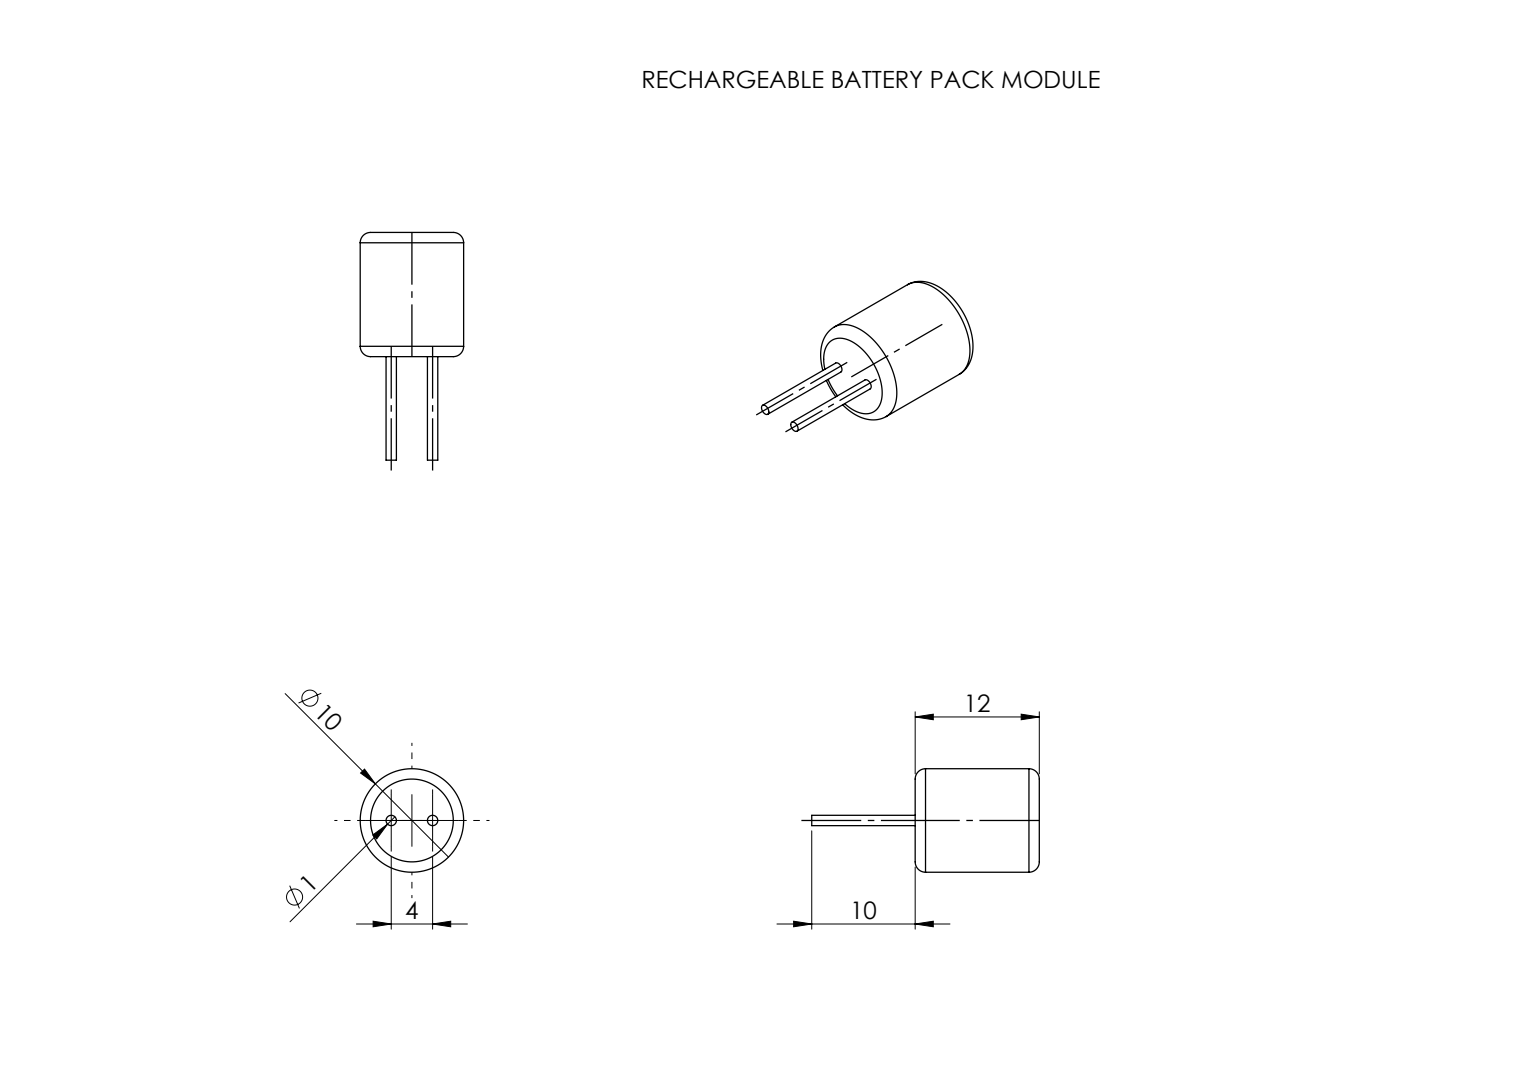
ISO-10303-21;
HEADER;
FILE_DESCRIPTION (('STEP AP214'),
    '1' );
FILE_NAME ('Rechargeable Battery Pack Module.step',
    '2026-10-02T09:26:43',
    ( '' ),
    ( '' ),
    'SwSTEP 2.0',
    'SolidWorks 2026',
    '' );
FILE_SCHEMA (( 'AUTOMOTIVE_DESIGN' ));
ENDSEC;

DATA;
#746=ORIENTED_EDGE ( 'NONE', *, *, #80621, .T. ) ;
#776=VERTEX_POINT ( 'NONE', #34676 ) ;
#917=CYLINDRICAL_SURFACE ( 'NONE', #50212, 0.5000000000000000000 ) ;
#1131=EDGE_LOOP ( 'NONE', ( #25952, #97783 ) ) ;
#1207=DIRECTION ( 'NONE',  ( -1.000000000000000000, -0.000000000000000000, -0.000000000000000000 ) ) ;
#1347=AXIS2_PLACEMENT_3D ( 'NONE', #82334, #73777, #14206 ) ;
#1619=AXIS2_PLACEMENT_3D ( 'NONE', #126509, #36204, #55191 ) ;
#1764=VERTEX_POINT ( 'NONE', #56391 ) ;
#1811=ORIENTED_EDGE ( 'NONE', *, *, #13485, .F. ) ;
#1941=CARTESIAN_POINT ( 'NONE',  ( 175.5000000000000000, 0.000000000000000000, 0.000000000000000000 ) ) ;
#2072=ORIENTED_EDGE ( 'NONE', *, *, #96533, .F. ) ;
#2393=ADVANCED_BREP_SHAPE_REPRESENTATION ( '', ( #58784, #108296 ), #47765 ) ;
#2982=FACE_OUTER_BOUND ( 'NONE', #6815, .T. ) ;
#3352=DIRECTION ( 'NONE',  ( 0.000000000000000000, 0.000000000000000000, 1.000000000000000000 ) ) ;
#3364=CARTESIAN_POINT ( 'NONE',  ( 175.5000000000000000, 0.000000000000000000, 0.000000000000000000 ) ) ;
#3537=EDGE_LOOP ( 'NONE', ( #83480, #102530 ) ) ;
#4172=AXIS2_PLACEMENT_3D ( 'NONE', #93028, #43934, #3352 ) ;
#4527=ORIENTED_EDGE ( 'NONE', *, *, #55775, .F. ) ;
#4887=CARTESIAN_POINT ( 'NONE',  ( 186.5000000000000000, 6.123233995736766282E-16, 5.000000000000000000 ) ) ;
#4950=DIRECTION ( 'NONE',  ( -1.000000000000000000, -0.000000000000000000, -0.000000000000000000 ) ) ;
#5196=CARTESIAN_POINT ( 'NONE',  ( 165.4999999999999716, 0.000000000000000000, -2.000000000000000000 ) ) ;
#5265=LINE ( 'NONE', #85119, #87555 ) ;
#5270=VERTEX_POINT ( 'NONE', #43477 ) ;
#5812=VERTEX_POINT ( 'NONE', #83730 ) ;
#5997=ADVANCED_FACE ( 'NONE', ( #126226, #56814, #26736 ), #106576, .F. ) ;
#6574=AXIS2_PLACEMENT_3D ( 'NONE', #103013, #82092, #70987 ) ;
#6622=ORIENTED_EDGE ( 'NONE', *, *, #108928, .T. ) ;
#6815=EDGE_LOOP ( 'NONE', ( #71189, #21105 ) ) ;
#6854=AXIS2_PLACEMENT_3D ( 'NONE', #39231, #123387, #33723 ) ;
#6983=CIRCLE ( 'NONE', #86415, 0.5000000000000000000 ) ;
#7177=DIRECTION ( 'NONE',  ( -1.000000000000000000, 0.000000000000000000, 0.000000000000000000 ) ) ;
#7523=DIRECTION ( 'NONE',  ( 0.000000000000000000, 0.000000000000000000, -1.000000000000000000 ) ) ;
#7960=DIRECTION ( 'NONE',  ( 0.000000000000000000, 0.000000000000000000, -1.000000000000000000 ) ) ;
#8623=EDGE_CURVE ( 'NONE', #119894, #23306, #120776, .T. ) ;
#8804=CARTESIAN_POINT ( 'NONE',  ( 187.5000000000000000, 0.000000000000000000, 0.000000000000000000 ) ) ;
#8811=CARTESIAN_POINT ( 'NONE',  ( 175.5000000000000000, 0.000000000000000000, 0.000000000000000000 ) ) ;
#9559=DIRECTION ( 'NONE',  ( 0.000000000000000000, -1.000000000000000000, 0.000000000000000000 ) ) ;
#9943=EDGE_CURVE ( 'NONE', #1764, #33342, #80190, .T. ) ;
#10096=DIRECTION ( 'NONE',  ( 0.000000000000000000, 0.000000000000000000, -1.000000000000000000 ) ) ;
#10644=CARTESIAN_POINT ( 'NONE',  ( 0.000000000000000000, 0.000000000000000000, 0.000000000000000000 ) ) ;
#10764=DIRECTION ( 'NONE',  ( 1.000000000000000000, -0.000000000000000000, -0.000000000000000000 ) ) ;
#10828=EDGE_CURVE ( 'NONE', #35122, #42109, #78651, .T. ) ;
#10998=EDGE_CURVE ( 'NONE', #33342, #119894, #56943, .T. ) ;
#11004=DIRECTION ( 'NONE',  ( 1.000000000000000000, 0.000000000000000000, 0.000000000000000000 ) ) ;
#11153=( NAMED_UNIT ( * ) PLANE_ANGLE_UNIT ( ) SI_UNIT ( $, .RADIAN. ) );
#11467=ADVANCED_FACE ( 'NONE', ( #2982 ), #43565, .T. ) ;
#11539=ORIENTED_EDGE ( 'NONE', *, *, #10998, .T. ) ;
#12671=CARTESIAN_POINT ( 'NONE',  ( 165.4999999999999716, 6.123233995736768501E-17, 2.500000000000000000 ) ) ;
#13485=EDGE_CURVE ( 'NONE', #33342, #41996, #5265, .T. ) ;
#13529=DIRECTION ( 'NONE',  ( 1.000000000000000000, -0.000000000000000000, -0.000000000000000000 ) ) ;
#13551=DIRECTION ( 'NONE',  ( 0.000000000000000000, 1.224646799147353454E-16, 1.000000000000000000 ) ) ;
#13811=CYLINDRICAL_SURFACE ( 'NONE', #120018, 5.000000000000000000 ) ;
#14206=DIRECTION ( 'NONE',  ( 0.000000000000000000, 0.000000000000000000, -1.000000000000000000 ) ) ;
#14451=DIRECTION ( 'NONE',  ( 0.000000000000000000, 0.000000000000000000, -1.000000000000000000 ) ) ;
#14818=PRODUCT_DEFINITION ( 'UNKNOWN', '', #92276, #105660 ) ;
#15075=VECTOR ( 'NONE', #28897, 1000.000000000000000 ) ;
#15705=DIRECTION ( 'NONE',  ( 0.000000000000000000, 0.000000000000000000, -1.000000000000000000 ) ) ;
#16006=CIRCLE ( 'NONE', #1347, 1.000000000000000000 ) ;
#16328=ORIENTED_EDGE ( 'NONE', *, *, #70791, .T. ) ;
#16423=( GEOMETRIC_REPRESENTATION_CONTEXT ( 3 ) GLOBAL_UNCERTAINTY_ASSIGNED_CONTEXT ( ( #128254 ) ) GLOBAL_UNIT_ASSIGNED_CONTEXT ( ( #21635, #43225, #83143 ) ) REPRESENTATION_CONTEXT ( 'NONE', 'WORKASPACE' ) );
#16594=EDGE_CURVE ( 'NONE', #35122, #21008, #121273, .T. ) ;
#16872=DIRECTION ( 'NONE',  ( 1.000000000000000000, 0.000000000000000000, 0.000000000000000000 ) ) ;
#17339=FACE_OUTER_BOUND ( 'NONE', #77583, .T. ) ;
#17709=SURFACE_STYLE_FILL_AREA ( #118495 ) ;
#17855=ORIENTED_EDGE ( 'NONE', *, *, #98166, .F. ) ;
#17906=ADVANCED_FACE ( 'NONE', ( #33015 ), #69295, .T. ) ;
#18275=UNCERTAINTY_MEASURE_WITH_UNIT (LENGTH_MEASURE( 1.000000000000000082E-05 ), #98248, 'distance_accuracy_value', 'NONE');
#18362=( LENGTH_UNIT ( ) NAMED_UNIT ( * ) SI_UNIT ( .MILLI., .METRE. ) );
#18958=DIRECTION ( 'NONE',  ( 1.000000000000000000, -0.000000000000000000, -0.000000000000000000 ) ) ;
#19275=ADVANCED_FACE ( 'NONE', ( #71652 ), #33040, .T. ) ;
#19624=CARTESIAN_POINT ( 'NONE',  ( 165.4999999999999716, 0.000000000000000000, -2.000000000000000000 ) ) ;
#19681=CARTESIAN_POINT ( 'NONE',  ( 187.5000000000000000, 0.000000000000000000, 0.000000000000000000 ) ) ;
#20983=SHAPE_REPRESENTATION_RELATIONSHIP ( 'NONE' , 'NONE' ,  #120523, #2393 ) ;
#21008=VERTEX_POINT ( 'NONE', #102729 ) ;
#21105=ORIENTED_EDGE ( 'NONE', *, *, #91309, .T. ) ;
#21443=AXIS2_PLACEMENT_3D ( 'NONE', #8811, #128638, #38976 ) ;
#21635=( LENGTH_UNIT ( ) NAMED_UNIT ( * ) SI_UNIT ( .MILLI., .METRE. ) );
#21971=CIRCLE ( 'NONE', #47098, 4.000000000000000000 ) ;
#22369=CIRCLE ( 'NONE', #39099, 4.000000000000000000 ) ;
#22997=DIRECTION ( 'NONE',  ( 1.000000000000000000, 0.000000000000000000, 0.000000000000000000 ) ) ;
#23306=VERTEX_POINT ( 'NONE', #4887 ) ;
#23888=CARTESIAN_POINT ( 'NONE',  ( 175.5000000000000000, 6.123233995736768501E-17, -1.500000000000000000 ) ) ;
#24106=AXIS2_PLACEMENT_3D ( 'NONE', #50924, #71851, #13551 ) ;
#24229=CARTESIAN_POINT ( 'NONE',  ( 165.4999999999999716, 0.000000000000000000, 2.000000000000000000 ) ) ;
#24376=EDGE_LOOP ( 'NONE', ( #35580, #95950 ) ) ;
#25759=DIRECTION ( 'NONE',  ( 0.000000000000000000, 0.000000000000000000, -1.000000000000000000 ) ) ;
#25952=ORIENTED_EDGE ( 'NONE', *, *, #89020, .F. ) ;
#26172=AXIS2_PLACEMENT_3D ( 'NONE', #58712, #116323, #125509 ) ;
#26308=CARTESIAN_POINT ( 'NONE',  ( 165.4999999999999716, 0.000000000000000000, 1.500000000000000000 ) ) ;
#26592=ORIENTED_EDGE ( 'NONE', *, *, #35766, .F. ) ;
#26736=FACE_OUTER_BOUND ( 'NONE', #3537, .T. ) ;
#27119=CARTESIAN_POINT ( 'NONE',  ( 176.5000000000000000, 4.898587196589412829E-16, 4.000000000000000000 ) ) ;
#27510=EDGE_CURVE ( 'NONE', #23306, #50259, #76339, .T. ) ;
#27671=AXIS2_PLACEMENT_3D ( 'NONE', #8804, #88675, #7523 ) ;
#28249=DIRECTION ( 'NONE',  ( 0.000000000000000000, 0.000000000000000000, -1.000000000000000000 ) ) ;
#28846=SURFACE_SIDE_STYLE ('',( #17709 ) ) ;
#28897=DIRECTION ( 'NONE',  ( 1.000000000000000000, -0.000000000000000000, -0.000000000000000000 ) ) ;
#29136=CYLINDRICAL_SURFACE ( 'NONE', #21443, 5.000000000000000000 ) ;
#29448=FACE_OUTER_BOUND ( 'NONE', #118119, .T. ) ;
#29486=( NAMED_UNIT ( * ) PLANE_ANGLE_UNIT ( ) SI_UNIT ( $, .RADIAN. ) );
#31525=ADVANCED_FACE ( 'NONE', ( #86216 ), #88858, .T. ) ;
#32767=FILL_AREA_STYLE ('',( #71356 ) ) ;
#33015=FACE_OUTER_BOUND ( 'NONE', #42591, .T. ) ;
#33040=CYLINDRICAL_SURFACE ( 'NONE', #103130, 0.5000000000000000000 ) ;
#33189=CLOSED_SHELL ( 'NONE', ( #78152, #101719, #106871, #17906, #59315, #34332, #5997, #94137, #31525, #99429, #19275, #64468, #61554, #11467 ) ) ;
#33342=VERTEX_POINT ( 'NONE', #84485 ) ;
#33422=DIRECTION ( 'NONE',  ( -0.000000000000000000, 0.000000000000000000, -1.000000000000000000 ) ) ;
#33562=EDGE_LOOP ( 'NONE', ( #120291, #124667, #73285, #26592 ) ) ;
#33723=DIRECTION ( 'NONE',  ( 0.000000000000000000, 0.000000000000000000, 1.000000000000000000 ) ) ;
#34063=EDGE_CURVE ( 'NONE', #776, #90572, #109164, .T. ) ;
#34332=ADVANCED_FACE ( 'NONE', ( #17339 ), #29136, .T. ) ;
#34676=CARTESIAN_POINT ( 'NONE',  ( 175.5000000000000000, 6.123233995736768501E-17, 2.500000000000000000 ) ) ;
#34933=ORIENTED_EDGE ( 'NONE', *, *, #9943, .F. ) ;
#35122=VERTEX_POINT ( 'NONE', #50236 ) ;
#35248=STYLED_ITEM ( 'NONE', ( #111273 ), #2393 ) ;
#35580=ORIENTED_EDGE ( 'NONE', *, *, #39365, .T. ) ;
#35766=EDGE_CURVE ( 'NONE', #50259, #74009, #61339, .T. ) ;
#35831=DIRECTION ( 'NONE',  ( -1.000000000000000000, -0.000000000000000000, -0.000000000000000000 ) ) ;
#36204=DIRECTION ( 'NONE',  ( -1.000000000000000000, -0.000000000000000000, -0.000000000000000000 ) ) ;
#36517=ORIENTED_EDGE ( 'NONE', *, *, #45709, .T. ) ;
#37749=AXIS2_PLACEMENT_3D ( 'NONE', #46198, #77579, #66477 ) ;
#37752=ORIENTED_EDGE ( 'NONE', *, *, #27510, .T. ) ;
#37900=ORIENTED_EDGE ( 'NONE', *, *, #124325, .T. ) ;
#38010=SURFACE_STYLE_USAGE ( .BOTH. , #28846 ) ;
#38195=AXIS2_PLACEMENT_3D ( 'NONE', #19624, #18958, #108639 ) ;
#38976=DIRECTION ( 'NONE',  ( 0.000000000000000000, 0.000000000000000000, -1.000000000000000000 ) ) ;
#39099=AXIS2_PLACEMENT_3D ( 'NONE', #19681, #79883, #129018 ) ;
#39231=CARTESIAN_POINT ( 'NONE',  ( 165.4999999999999716, 0.000000000000000000, -2.000000000000000000 ) ) ;
#39365=EDGE_CURVE ( 'NONE', #74009, #50259, #22369, .T. ) ;
#41996=VERTEX_POINT ( 'NONE', #81916 ) ;
#42012=AXIS2_PLACEMENT_3D ( 'NONE', #24229, #122438, #33422 ) ;
#42109=VERTEX_POINT ( 'NONE', #65498 ) ;
#42591=EDGE_LOOP ( 'NONE', ( #42743, #37752, #115653, #17855 ) ) ;
#42743=ORIENTED_EDGE ( 'NONE', *, *, #122243, .F. ) ;
#43225=( NAMED_UNIT ( * ) PLANE_ANGLE_UNIT ( ) SI_UNIT ( $, .RADIAN. ) );
#43477=CARTESIAN_POINT ( 'NONE',  ( 175.5000000000000000, 5.510910596163088569E-16, 4.000000000000000000 ) ) ;
#43565=PLANE ( 'NONE',  #6854 ) ;
#43718=AXIS2_PLACEMENT_3D ( 'NONE', #94933, #7177, #15705 ) ;
#43934=DIRECTION ( 'NONE',  ( -1.000000000000000000, 0.000000000000000000, 0.000000000000000000 ) ) ;
#44859=CARTESIAN_POINT ( 'NONE',  ( 186.5000000000000000, 0.000000000000000000, 0.000000000000000000 ) ) ;
#45113=CARTESIAN_POINT ( 'NONE',  ( 187.5000000000000000, 0.000000000000000000, -4.000000000000000000 ) ) ;
#45709=EDGE_CURVE ( 'NONE', #50667, #42109, #55992, .T. ) ;
#45841=LINE ( 'NONE', #125666, #52947 ) ;
#45939=DIRECTION ( 'NONE',  ( -1.000000000000000000, -0.000000000000000000, -0.000000000000000000 ) ) ;
#46198=CARTESIAN_POINT ( 'NONE',  ( 175.5000000000000000, 0.000000000000000000, -2.000000000000000000 ) ) ;
#47098=AXIS2_PLACEMENT_3D ( 'NONE', #96947, #45939, #106135 ) ;
#47415=VECTOR ( 'NONE', #54414, 1000.000000000000000 ) ;
#47554=DIRECTION ( 'NONE',  ( 0.000000000000000000, 0.000000000000000000, -1.000000000000000000 ) ) ;
#47765=( GEOMETRIC_REPRESENTATION_CONTEXT ( 3 ) GLOBAL_UNCERTAINTY_ASSIGNED_CONTEXT ( ( #18275 ) ) GLOBAL_UNIT_ASSIGNED_CONTEXT ( ( #98248, #11153, #111956 ) ) REPRESENTATION_CONTEXT ( 'NONE', 'WORKASPACE' ) );
#47900=CARTESIAN_POINT ( 'NONE',  ( 176.5000000000000000, 0.000000000000000000, 0.000000000000000000 ) ) ;
#50212=AXIS2_PLACEMENT_3D ( 'NONE', #51968, #101707, #10096 ) ;
#50236=CARTESIAN_POINT ( 'NONE',  ( 165.4999999999999716, 0.000000000000000000, -2.500000000000000000 ) ) ;
#50259=VERTEX_POINT ( 'NONE', #124475 ) ;
#50440=SURFACE_SIDE_STYLE ('',( #70094 ) ) ;
#50555=VECTOR ( 'NONE', #72338, 1000.000000000000000 ) ;
#50667=VERTEX_POINT ( 'NONE', #23888 ) ;
#50873=COLOUR_RGB ( '', 0.08235294, 0.09019608, 0.10196078) ;
#50924=CARTESIAN_POINT ( 'NONE',  ( 186.5000000000000000, 4.898587196589412829E-16, 4.000000000000000000 ) ) ;
#51034=CYLINDRICAL_SURFACE ( 'NONE', #38195, 0.5000000000000000000 ) ;
#51417=CARTESIAN_POINT ( 'NONE',  ( 175.5000000000000000, 6.123233995736766282E-16, 5.000000000000000000 ) ) ;
#51968=CARTESIAN_POINT ( 'NONE',  ( 165.4999999999999716, 0.000000000000000000, 2.000000000000000000 ) ) ;
#52127=EDGE_LOOP ( 'NONE', ( #98198, #121992 ) ) ;
#52397=PRODUCT ( 'Rechargeable Battery Pack Module', 'Rechargeable Battery Pack Module', '', ( #107919 ) ) ;
#52947=VECTOR ( 'NONE', #88145, 1000.000000000000000 ) ;
#54111=CARTESIAN_POINT ( 'NONE',  ( 165.4999999999999716, 0.000000000000000000, -2.000000000000000000 ) ) ;
#54316=DIRECTION ( 'NONE',  ( 0.000000000000000000, 0.000000000000000000, 1.000000000000000000 ) ) ;
#54414=DIRECTION ( 'NONE',  ( 1.000000000000000000, -0.000000000000000000, -0.000000000000000000 ) ) ;
#54895=ORIENTED_EDGE ( 'NONE', *, *, #89020, .T. ) ;
#55191=DIRECTION ( 'NONE',  ( 0.000000000000000000, 0.000000000000000000, -1.000000000000000000 ) ) ;
#55775=EDGE_CURVE ( 'NONE', #5270, #1764, #21971, .T. ) ;
#55992=CIRCLE ( 'NONE', #1619, 0.5000000000000000000 ) ;
#56335=APPLICATION_CONTEXT ( 'automotive_design' ) ;
#56391=CARTESIAN_POINT ( 'NONE',  ( 175.5000000000000000, 0.000000000000000000, -4.000000000000000000 ) ) ;
#56814=FACE_BOUND ( 'NONE', #1131, .T. ) ;
#56943=CIRCLE ( 'NONE', #104977, 5.000000000000000000 ) ;
#57565=CIRCLE ( 'NONE', #74287, 5.000000000000000000 ) ;
#58263=ORIENTED_EDGE ( 'NONE', *, *, #10828, .F. ) ;
#58296=EDGE_LOOP ( 'NONE', ( #128153, #2072, #97662, #116249 ) ) ;
#58712=CARTESIAN_POINT ( 'NONE',  ( 186.5000000000000000, 0.000000000000000000, 0.000000000000000000 ) ) ;
#58784=MANIFOLD_SOLID_BREP ( 'Boss-Extrude2', #33189 ) ;
#59084=CARTESIAN_POINT ( 'NONE',  ( 176.5000000000000000, 0.000000000000000000, 0.000000000000000000 ) ) ;
#59315=ADVANCED_FACE ( 'NONE', ( #93678 ), #13811, .T. ) ;
#59615=( NAMED_UNIT ( * ) SI_UNIT ( $, .STERADIAN. ) SOLID_ANGLE_UNIT ( ) );
#59872=FACE_OUTER_BOUND ( 'NONE', #114198, .T. ) ;
#59899=AXIS2_PLACEMENT_3D ( 'NONE', #119083, #128272, #118427 ) ;
#60259=ORIENTED_EDGE ( 'NONE', *, *, #16594, .F. ) ;
#60304=DIRECTION ( 'NONE',  ( 0.000000000000000000, 0.000000000000000000, -1.000000000000000000 ) ) ;
#60409=ORIENTED_EDGE ( 'NONE', *, *, #90299, .T. ) ;
#60774=FACE_OUTER_BOUND ( 'NONE', #58296, .T. ) ;
#60789=AXIS2_PLACEMENT_3D ( 'NONE', #109866, #71217, #89573 ) ;
#61158=EDGE_CURVE ( 'NONE', #105300, #776, #73409, .T. ) ;
#61339=CIRCLE ( 'NONE', #124025, 4.000000000000000000 ) ;
#61554=ADVANCED_FACE ( 'NONE', ( #81628 ), #92756, .T. ) ;
#62488=CIRCLE ( 'NONE', #43718, 0.5000000000000000000 ) ;
#63763=DIRECTION ( 'NONE',  ( 1.000000000000000000, 0.000000000000000000, 0.000000000000000000 ) ) ;
#63773=ORIENTED_EDGE ( 'NONE', *, *, #87513, .F. ) ;
#64468=ADVANCED_FACE ( 'NONE', ( #83162 ), #73314, .F. ) ;
#64769=DIRECTION ( 'NONE',  ( -1.000000000000000000, 0.000000000000000000, 0.000000000000000000 ) ) ;
#65498=CARTESIAN_POINT ( 'NONE',  ( 175.5000000000000000, 0.000000000000000000, -2.500000000000000000 ) ) ;
#65742=DIRECTION ( 'NONE',  ( 0.000000000000000000, 1.000000000000000000, -1.224646799147353207E-16 ) ) ;
#65808=CARTESIAN_POINT ( 'NONE',  ( 175.5000000000000000, 0.000000000000000000, 2.000000000000000000 ) ) ;
#66477=DIRECTION ( 'NONE',  ( 0.000000000000000000, 0.000000000000000000, -1.000000000000000000 ) ) ;
#66646=CARTESIAN_POINT ( 'NONE',  ( 175.5000000000000000, 0.000000000000000000, 0.000000000000000000 ) ) ;
#66719=ORIENTED_EDGE ( 'NONE', *, *, #61158, .F. ) ;
#67436=FILL_AREA_STYLE_COLOUR ( '', #50873 ) ;
#67598=ORIENTED_EDGE ( 'NONE', *, *, #108928, .F. ) ;
#68414=AXIS2_PLACEMENT_3D ( 'NONE', #54111, #13529, #121547 ) ;
#69295=TOROIDAL_SURFACE ( 'NONE', #6574, 4.000000000000000000, 1.000000000000000000 ) ;
#69442=CARTESIAN_POINT ( 'NONE',  ( 176.5000000000000000, 0.000000000000000000, 0.000000000000000000 ) ) ;
#70045=ORIENTED_EDGE ( 'NONE', *, *, #10998, .F. ) ;
#70094=SURFACE_STYLE_FILL_AREA ( #32767 ) ;
#70791=EDGE_CURVE ( 'NONE', #5270, #119894, #99880, .T. ) ;
#70987=DIRECTION ( 'NONE',  ( 0.000000000000000000, 0.000000000000000000, -1.000000000000000000 ) ) ;
#71189=ORIENTED_EDGE ( 'NONE', *, *, #16594, .T. ) ;
#71217=DIRECTION ( 'NONE',  ( -1.000000000000000000, 0.000000000000000000, 0.000000000000000000 ) ) ;
#71356=FILL_AREA_STYLE_COLOUR ( '', #120907 ) ;
#71652=FACE_OUTER_BOUND ( 'NONE', #76742, .T. ) ;
#71851=DIRECTION ( 'NONE',  ( 0.000000000000000000, 1.000000000000000000, -1.224646799147353207E-16 ) ) ;
#72338=DIRECTION ( 'NONE',  ( 1.000000000000000000, 0.000000000000000000, 0.000000000000000000 ) ) ;
#72946=CARTESIAN_POINT ( 'NONE',  ( 165.4999999999999716, 0.000000000000000000, 2.000000000000000000 ) ) ;
#73285=ORIENTED_EDGE ( 'NONE', *, *, #98166, .T. ) ;
#73314=PLANE ( 'NONE',  #42012 ) ;
#73409=LINE ( 'NONE', #97406, #47415 ) ;
#73777=DIRECTION ( 'NONE',  ( 0.000000000000000000, -1.000000000000000000, 0.000000000000000000 ) ) ;
#74009=VERTEX_POINT ( 'NONE', #45113 ) ;
#74287=AXIS2_PLACEMENT_3D ( 'NONE', #117247, #1207, #7960 ) ;
#75892=ORIENTED_EDGE ( 'NONE', *, *, #13485, .T. ) ;
#76339=CIRCLE ( 'NONE', #24106, 1.000000000000000000 ) ;
#76742=EDGE_LOOP ( 'NONE', ( #66719, #63773, #746, #54895 ) ) ;
#77579=DIRECTION ( 'NONE',  ( -1.000000000000000000, -0.000000000000000000, -0.000000000000000000 ) ) ;
#77583=EDGE_LOOP ( 'NONE', ( #113598, #113060, #75892, #99101 ) ) ;
#78152=ADVANCED_FACE ( 'NONE', ( #29448 ), #51034, .T. ) ;
#78651=LINE ( 'NONE', #118545, #15075 ) ;
#78757=ORIENTED_EDGE ( 'NONE', *, *, #91309, .F. ) ;
#79133=EDGE_LOOP ( 'NONE', ( #89365, #60409 ) ) ;
#79883=DIRECTION ( 'NONE',  ( 1.000000000000000000, 0.000000000000000000, 0.000000000000000000 ) ) ;
#80190=CIRCLE ( 'NONE', #96340, 1.000000000000000000 ) ;
#80621=EDGE_CURVE ( 'NONE', #5812, #90572, #128389, .T. ) ;
#80718=DIRECTION ( 'NONE',  ( 1.000000000000000000, 0.000000000000000000, 0.000000000000000000 ) ) ;
#81205=SURFACE_STYLE_USAGE ( .BOTH. , #50440 ) ;
#81298=CIRCLE ( 'NONE', #100083, 5.000000000000000000 ) ;
#81628=FACE_OUTER_BOUND ( 'NONE', #81771, .T. ) ;
#81771=EDGE_LOOP ( 'NONE', ( #67598, #60259, #104867, #37900 ) ) ;
#81916=CARTESIAN_POINT ( 'NONE',  ( 186.5000000000000000, 0.000000000000000000, -5.000000000000000000 ) ) ;
#82092=DIRECTION ( 'NONE',  ( 1.000000000000000000, 0.000000000000000000, 0.000000000000000000 ) ) ;
#82177=MECHANICAL_DESIGN_GEOMETRIC_PRESENTATION_REPRESENTATION('',(#124026),#90576);
#82334=CARTESIAN_POINT ( 'NONE',  ( 186.5000000000000000, 0.000000000000000000, -4.000000000000000000 ) ) ;
#83143=( NAMED_UNIT ( * ) SI_UNIT ( $, .STERADIAN. ) SOLID_ANGLE_UNIT ( ) );
#83162=FACE_OUTER_BOUND ( 'NONE', #79133, .T. ) ;
#83480=ORIENTED_EDGE ( 'NONE', *, *, #96533, .T. ) ;
#83660=EDGE_LOOP ( 'NONE', ( #4527, #16328, #70045, #34933 ) ) ;
#83730=CARTESIAN_POINT ( 'NONE',  ( 165.4999999999999716, 0.000000000000000000, 1.500000000000000000 ) ) ;
#83768=CIRCLE ( 'NONE', #60789, 0.5000000000000000000 ) ;
#84485=CARTESIAN_POINT ( 'NONE',  ( 176.5000000000000000, 0.000000000000000000, -5.000000000000000000 ) ) ;
#84996=CIRCLE ( 'NONE', #59899, 5.000000000000000000 ) ;
#85119=CARTESIAN_POINT ( 'NONE',  ( 175.5000000000000000, 0.000000000000000000, -5.000000000000000000 ) ) ;
#85442=AXIS2_PLACEMENT_3D ( 'NONE', #66646, #16872, #96746 ) ;
#86216=FACE_OUTER_BOUND ( 'NONE', #33562, .T. ) ;
#86415=AXIS2_PLACEMENT_3D ( 'NONE', #86856, #35831, #125492 ) ;
#86856=CARTESIAN_POINT ( 'NONE',  ( 175.5000000000000000, 0.000000000000000000, 2.000000000000000000 ) ) ;
#87333=AXIS2_PLACEMENT_3D ( 'NONE', #27119, #65742, #105683 ) ;
#87513=EDGE_CURVE ( 'NONE', #5812, #105300, #83768, .T. ) ;
#87555=VECTOR ( 'NONE', #22997, 1000.000000000000000 ) ;
#88001=PLANE ( 'NONE',  #27671 ) ;
#88145=DIRECTION ( 'NONE',  ( 1.000000000000000000, -0.000000000000000000, -0.000000000000000000 ) ) ;
#88244=TOROIDAL_SURFACE ( 'NONE', #123752, 4.000000000000000000, 1.000000000000000000 ) ;
#88675=DIRECTION ( 'NONE',  ( 1.000000000000000000, 0.000000000000000000, 0.000000000000000000 ) ) ;
#88858=TOROIDAL_SURFACE ( 'NONE', #26172, 4.000000000000000000, 1.000000000000000000 ) ;
#89020=EDGE_CURVE ( 'NONE', #90572, #776, #6983, .T. ) ;
#89073=AXIS2_PLACEMENT_3D ( 'NONE', #1941, #121085, #113185 ) ;
#89365=ORIENTED_EDGE ( 'NONE', *, *, #87513, .T. ) ;
#89573=DIRECTION ( 'NONE',  ( 0.000000000000000000, 0.000000000000000000, -1.000000000000000000 ) ) ;
#90299=EDGE_CURVE ( 'NONE', #105300, #5812, #62488, .T. ) ;
#90516=DIRECTION ( 'NONE',  ( 0.000000000000000000, 0.000000000000000000, 1.000000000000000000 ) ) ;
#90572=VERTEX_POINT ( 'NONE', #119715 ) ;
#90576=( GEOMETRIC_REPRESENTATION_CONTEXT ( 3 ) GLOBAL_UNCERTAINTY_ASSIGNED_CONTEXT ( ( #103088 ) ) GLOBAL_UNIT_ASSIGNED_CONTEXT ( ( #18362, #29486, #59615 ) ) REPRESENTATION_CONTEXT ( 'NONE', 'WORKASPACE' ) );
#91309=EDGE_CURVE ( 'NONE', #21008, #35122, #127595, .T. ) ;
#91941=DIRECTION ( 'NONE',  ( 0.000000000000000000, 0.000000000000000000, -1.000000000000000000 ) ) ;
#92096=PRODUCT_DEFINITION_SHAPE ( 'NONE', 'NONE',  #14818 ) ;
#92276=PRODUCT_DEFINITION_FORMATION_WITH_SPECIFIED_SOURCE ( 'ANY', '', #52397, .NOT_KNOWN. ) ;
#92756=CYLINDRICAL_SURFACE ( 'NONE', #68414, 0.5000000000000000000 ) ;
#93028=CARTESIAN_POINT ( 'NONE',  ( 165.4999999999999716, 0.000000000000000000, -2.000000000000000000 ) ) ;
#93678=FACE_OUTER_BOUND ( 'NONE', #93694, .T. ) ;
#93694=EDGE_LOOP ( 'NONE', ( #11539, #115976, #120469, #1811 ) ) ;
#94137=ADVANCED_FACE ( 'NONE', ( #127951 ), #88001, .T. ) ;
#94306=DIRECTION ( 'NONE',  ( 1.000000000000000000, 0.000000000000000000, 0.000000000000000000 ) ) ;
#94933=CARTESIAN_POINT ( 'NONE',  ( 165.4999999999999716, 0.000000000000000000, 2.000000000000000000 ) ) ;
#95883=DIRECTION ( 'NONE',  ( -1.000000000000000000, -0.000000000000000000, -0.000000000000000000 ) ) ;
#95950=ORIENTED_EDGE ( 'NONE', *, *, #35766, .T. ) ;
#96184=AXIS2_PLACEMENT_3D ( 'NONE', #5196, #64769, #54316 ) ;
#96340=AXIS2_PLACEMENT_3D ( 'NONE', #127400, #9559, #47554 ) ;
#96533=EDGE_CURVE ( 'NONE', #1764, #5270, #114106, .T. ) ;
#96746=DIRECTION ( 'NONE',  ( 0.000000000000000000, 0.000000000000000000, -1.000000000000000000 ) ) ;
#96947=CARTESIAN_POINT ( 'NONE',  ( 175.5000000000000000, 0.000000000000000000, 0.000000000000000000 ) ) ;
#97406=CARTESIAN_POINT ( 'NONE',  ( 165.4999999999999716, 6.123233995736767268E-17, 2.500000000000000000 ) ) ;
#97543=ORIENTED_EDGE ( 'NONE', *, *, #34063, .T. ) ;
#97662=ORIENTED_EDGE ( 'NONE', *, *, #9943, .T. ) ;
#97783=ORIENTED_EDGE ( 'NONE', *, *, #34063, .F. ) ;
#98166=EDGE_CURVE ( 'NONE', #41996, #74009, #16006, .T. ) ;
#98198=ORIENTED_EDGE ( 'NONE', *, *, #124325, .F. ) ;
#98248=( LENGTH_UNIT ( ) NAMED_UNIT ( * ) SI_UNIT ( .MILLI., .METRE. ) );
#98361=CIRCLE ( 'NONE', #37749, 0.5000000000000000000 ) ;
#99101=ORIENTED_EDGE ( 'NONE', *, *, #116547, .T. ) ;
#99429=ADVANCED_FACE ( 'NONE', ( #60774 ), #112549, .T. ) ;
#99880=CIRCLE ( 'NONE', #87333, 1.000000000000000000 ) ;
#99957=ORIENTED_EDGE ( 'NONE', *, *, #80621, .F. ) ;
#100083=AXIS2_PLACEMENT_3D ( 'NONE', #44859, #95883, #115496 ) ;
#101707=DIRECTION ( 'NONE',  ( 1.000000000000000000, -0.000000000000000000, -0.000000000000000000 ) ) ;
#101719=ADVANCED_FACE ( 'NONE', ( #59872 ), #917, .T. ) ;
#102530=ORIENTED_EDGE ( 'NONE', *, *, #55775, .T. ) ;
#102729=CARTESIAN_POINT ( 'NONE',  ( 165.4999999999999716, 6.123233995736768501E-17, -1.500000000000000000 ) ) ;
#103013=CARTESIAN_POINT ( 'NONE',  ( 186.5000000000000000, 0.000000000000000000, 0.000000000000000000 ) ) ;
#103088=UNCERTAINTY_MEASURE_WITH_UNIT (LENGTH_MEASURE( 1.000000000000000082E-05 ), #18362, 'distance_accuracy_value', 'NONE');
#103130=AXIS2_PLACEMENT_3D ( 'NONE', #72946, #10764, #91941 ) ;
#104867=ORIENTED_EDGE ( 'NONE', *, *, #10828, .T. ) ;
#104977=AXIS2_PLACEMENT_3D ( 'NONE', #69442, #110033, #60304 ) ;
#105300=VERTEX_POINT ( 'NONE', #12671 ) ;
#105361=ORIENTED_EDGE ( 'NONE', *, *, #90299, .F. ) ;
#105660=PRODUCT_DEFINITION_CONTEXT ( 'detailed design', #114080, 'design' ) ;
#105683=DIRECTION ( 'NONE',  ( 0.000000000000000000, 1.224646799147353454E-16, 1.000000000000000000 ) ) ;
#106135=DIRECTION ( 'NONE',  ( 0.000000000000000000, 0.000000000000000000, -1.000000000000000000 ) ) ;
#106576=PLANE ( 'NONE',  #85442 ) ;
#106871=ADVANCED_FACE ( 'NONE', ( #112048 ), #88244, .T. ) ;
#107919=PRODUCT_CONTEXT ( 'NONE', #56335, 'mechanical' ) ;
#108071=DIRECTION ( 'NONE',  ( 1.000000000000000000, -0.000000000000000000, -0.000000000000000000 ) ) ;
#108296=AXIS2_PLACEMENT_3D ( 'NONE', #10644, #90516, #80718 ) ;
#108639=DIRECTION ( 'NONE',  ( 0.000000000000000000, 0.000000000000000000, -1.000000000000000000 ) ) ;
#108928=EDGE_CURVE ( 'NONE', #21008, #50667, #45841, .T. ) ;
#109164=CIRCLE ( 'NONE', #113384, 0.5000000000000000000 ) ;
#109866=CARTESIAN_POINT ( 'NONE',  ( 165.4999999999999716, 0.000000000000000000, 2.000000000000000000 ) ) ;
#110033=DIRECTION ( 'NONE',  ( 1.000000000000000000, 0.000000000000000000, 0.000000000000000000 ) ) ;
#110111=DIRECTION ( 'NONE',  ( 0.000000000000000000, 0.000000000000000000, -1.000000000000000000 ) ) ;
#111273=PRESENTATION_STYLE_ASSIGNMENT (( #81205 ) ) ;
#111956=( NAMED_UNIT ( * ) SI_UNIT ( $, .STERADIAN. ) SOLID_ANGLE_UNIT ( ) );
#112048=FACE_OUTER_BOUND ( 'NONE', #83660, .T. ) ;
#112549=TOROIDAL_SURFACE ( 'NONE', #120849, 4.000000000000000000, 1.000000000000000000 ) ;
#113060=ORIENTED_EDGE ( 'NONE', *, *, #118280, .T. ) ;
#113185=DIRECTION ( 'NONE',  ( 0.000000000000000000, 0.000000000000000000, -1.000000000000000000 ) ) ;
#113384=AXIS2_PLACEMENT_3D ( 'NONE', #65808, #4950, #125389 ) ;
#113598=ORIENTED_EDGE ( 'NONE', *, *, #8623, .F. ) ;
#114080=APPLICATION_CONTEXT ( 'automotive_design' ) ;
#114106=CIRCLE ( 'NONE', #89073, 4.000000000000000000 ) ;
#114146=CARTESIAN_POINT ( 'NONE',  ( 187.5000000000000000, 0.000000000000000000, 0.000000000000000000 ) ) ;
#114198=EDGE_LOOP ( 'NONE', ( #105361, #120710, #97543, #99957 ) ) ;
#115496=DIRECTION ( 'NONE',  ( 0.000000000000000000, 0.000000000000000000, -1.000000000000000000 ) ) ;
#115653=ORIENTED_EDGE ( 'NONE', *, *, #39365, .F. ) ;
#115976=ORIENTED_EDGE ( 'NONE', *, *, #8623, .T. ) ;
#116249=ORIENTED_EDGE ( 'NONE', *, *, #118280, .F. ) ;
#116323=DIRECTION ( 'NONE',  ( 1.000000000000000000, 0.000000000000000000, 0.000000000000000000 ) ) ;
#116547=EDGE_CURVE ( 'NONE', #41996, #23306, #57565, .T. ) ;
#117077=SHAPE_DEFINITION_REPRESENTATION ( #92096, #120523 ) ;
#117247=CARTESIAN_POINT ( 'NONE',  ( 186.5000000000000000, 0.000000000000000000, 0.000000000000000000 ) ) ;
#118119=EDGE_LOOP ( 'NONE', ( #78757, #6622, #36517, #58263 ) ) ;
#118280=EDGE_CURVE ( 'NONE', #119894, #33342, #84996, .T. ) ;
#118427=DIRECTION ( 'NONE',  ( 0.000000000000000000, 0.000000000000000000, -1.000000000000000000 ) ) ;
#118495=FILL_AREA_STYLE ('',( #67436 ) ) ;
#118545=CARTESIAN_POINT ( 'NONE',  ( 165.4999999999999716, 0.000000000000000000, -2.500000000000000000 ) ) ;
#119083=CARTESIAN_POINT ( 'NONE',  ( 176.5000000000000000, 0.000000000000000000, 0.000000000000000000 ) ) ;
#119715=CARTESIAN_POINT ( 'NONE',  ( 175.5000000000000000, 0.000000000000000000, 1.500000000000000000 ) ) ;
#119894=VERTEX_POINT ( 'NONE', #120169 ) ;
#120018=AXIS2_PLACEMENT_3D ( 'NONE', #3364, #94306, #14451 ) ;
#120169=CARTESIAN_POINT ( 'NONE',  ( 176.5000000000000000, 6.123233995736766282E-16, 5.000000000000000000 ) ) ;
#120291=ORIENTED_EDGE ( 'NONE', *, *, #27510, .F. ) ;
#120469=ORIENTED_EDGE ( 'NONE', *, *, #122243, .T. ) ;
#120523=SHAPE_REPRESENTATION ( 'Rechargeable Battery Pack Module', ( #108296 ), #47765 ) ;
#120710=ORIENTED_EDGE ( 'NONE', *, *, #61158, .T. ) ;
#120776=LINE ( 'NONE', #51417, #50555 ) ;
#120849=AXIS2_PLACEMENT_3D ( 'NONE', #47900, #11004, #28249 ) ;
#120907=COLOUR_RGB ( '', 0.08235294, 0.09019608, 0.10196078) ;
#121085=DIRECTION ( 'NONE',  ( -1.000000000000000000, -0.000000000000000000, -0.000000000000000000 ) ) ;
#121273=CIRCLE ( 'NONE', #4172, 0.5000000000000000000 ) ;
#121547=DIRECTION ( 'NONE',  ( 0.000000000000000000, 0.000000000000000000, -1.000000000000000000 ) ) ;
#121992=ORIENTED_EDGE ( 'NONE', *, *, #45709, .F. ) ;
#122243=EDGE_CURVE ( 'NONE', #23306, #41996, #81298, .T. ) ;
#122438=DIRECTION ( 'NONE',  ( 1.000000000000000000, 0.000000000000000000, -0.000000000000000000 ) ) ;
#122504=VECTOR ( 'NONE', #108071, 1000.000000000000000 ) ;
#123387=DIRECTION ( 'NONE',  ( -1.000000000000000000, 0.000000000000000000, 0.000000000000000000 ) ) ;
#123752=AXIS2_PLACEMENT_3D ( 'NONE', #59084, #129135, #110111 ) ;
#124025=AXIS2_PLACEMENT_3D ( 'NONE', #114146, #63763, #25759 ) ;
#124026=STYLED_ITEM ( 'NONE', ( #129001 ), #58784 ) ;
#124325=EDGE_CURVE ( 'NONE', #42109, #50667, #98361, .T. ) ;
#124475=CARTESIAN_POINT ( 'NONE',  ( 187.5000000000000000, 5.510910596163088569E-16, 4.000000000000000000 ) ) ;
#124667=ORIENTED_EDGE ( 'NONE', *, *, #116547, .F. ) ;
#125389=DIRECTION ( 'NONE',  ( 0.000000000000000000, 0.000000000000000000, -1.000000000000000000 ) ) ;
#125492=DIRECTION ( 'NONE',  ( 0.000000000000000000, 0.000000000000000000, -1.000000000000000000 ) ) ;
#125509=DIRECTION ( 'NONE',  ( 0.000000000000000000, 0.000000000000000000, -1.000000000000000000 ) ) ;
#125666=CARTESIAN_POINT ( 'NONE',  ( 165.4999999999999716, 6.123233995736767268E-17, -1.500000000000000000 ) ) ;
#126226=FACE_BOUND ( 'NONE', #52127, .T. ) ;
#126509=CARTESIAN_POINT ( 'NONE',  ( 175.5000000000000000, 0.000000000000000000, -2.000000000000000000 ) ) ;
#127400=CARTESIAN_POINT ( 'NONE',  ( 176.5000000000000000, 0.000000000000000000, -4.000000000000000000 ) ) ;
#127595=CIRCLE ( 'NONE', #96184, 0.5000000000000000000 ) ;
#127951=FACE_OUTER_BOUND ( 'NONE', #24376, .T. ) ;
#128153=ORIENTED_EDGE ( 'NONE', *, *, #70791, .F. ) ;
#128254=UNCERTAINTY_MEASURE_WITH_UNIT (LENGTH_MEASURE( 1.000000000000000082E-05 ), #21635, 'distance_accuracy_value', 'NONE');
#128272=DIRECTION ( 'NONE',  ( 1.000000000000000000, 0.000000000000000000, 0.000000000000000000 ) ) ;
#128389=LINE ( 'NONE', #26308, #122504 ) ;
#128638=DIRECTION ( 'NONE',  ( 1.000000000000000000, 0.000000000000000000, 0.000000000000000000 ) ) ;
#129001=PRESENTATION_STYLE_ASSIGNMENT (( #38010 ) ) ;
#129018=DIRECTION ( 'NONE',  ( 0.000000000000000000, 0.000000000000000000, -1.000000000000000000 ) ) ;
#129135=DIRECTION ( 'NONE',  ( 1.000000000000000000, 0.000000000000000000, 0.000000000000000000 ) ) ;
#129353=MECHANICAL_DESIGN_GEOMETRIC_PRESENTATION_REPRESENTATION('',(#35248),#16423);
ENDSEC;
END-ISO-10303-21;
